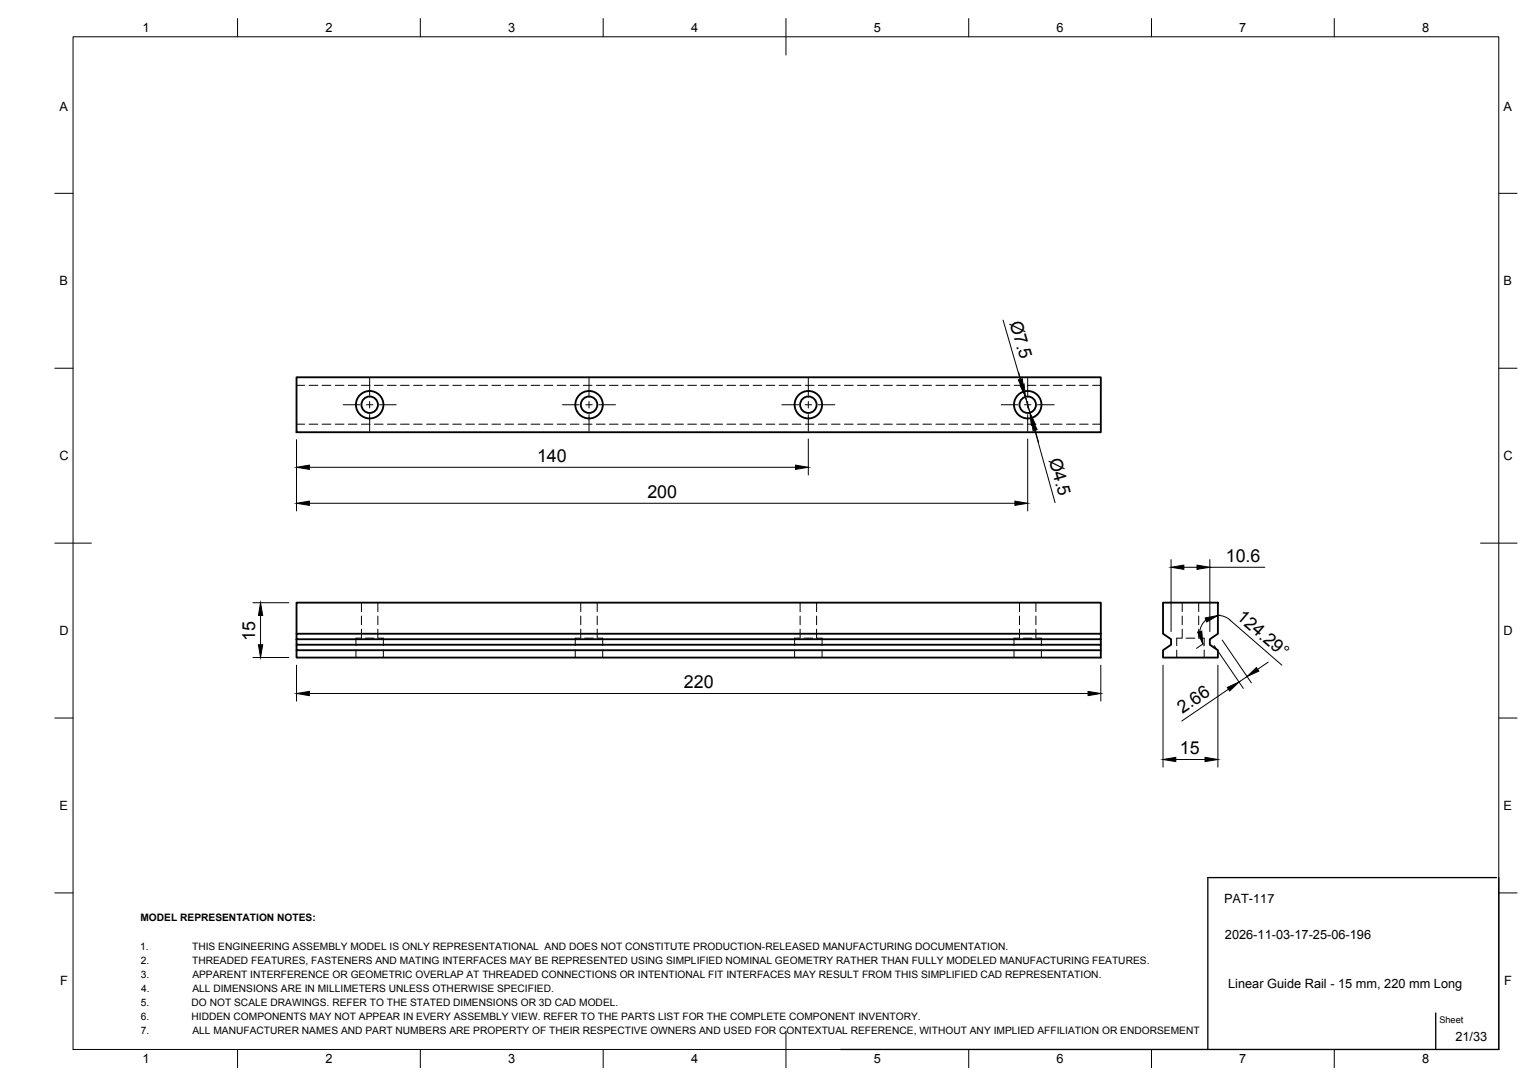
ISO-10303-21;
HEADER;
/* Generated by software containing ST-Developer
 * from STEP Tools, Inc. (www.steptools.com) 
 */

FILE_DESCRIPTION(
/* description */ ('Counterbalanced vertical column'),
/* implementation_level */ '2;1');

FILE_NAME(
/* name */ 'Linear Guide Rail - 15 mm, 220 mm Long.step',
/* time_stamp */ '2026-10-29T16:47:22-07:00',
/* author */ (''),
/* organization */ (''),
/* preprocessor_version */ 'ST-DEVELOPER v20.2',
/* originating_system */ 'Autodesk Translation Framework v15.17.0.0',
/* authorisation */ '');

FILE_SCHEMA (('AUTOMOTIVE_DESIGN { 1 0 10303 214 3 1 1 }'));
ENDSEC;

DATA;
#10=MECHANICAL_DESIGN_GEOMETRIC_PRESENTATION_REPRESENTATION('',(#368),#15040);
#298=SHAPE_REPRESENTATION_RELATIONSHIP('SRR','None',#15202,#333);
#333=ADVANCED_BREP_SHAPE_REPRESENTATION('',(#403),#15021);
#368=STYLED_ITEM('',(#15450),#403);
#403=MANIFOLD_SOLID_BREP('Body1',#7091);
#480=FACE_BOUND('',#1480,.T.);
#481=FACE_BOUND('',#1483,.T.);
#482=FACE_BOUND('',#1486,.T.);
#483=FACE_BOUND('',#1489,.T.);
#484=FACE_BOUND('',#1499,.T.);
#485=FACE_BOUND('',#1500,.T.);
#486=FACE_BOUND('',#1501,.T.);
#487=FACE_BOUND('',#1502,.T.);
#488=FACE_BOUND('',#1509,.T.);
#489=FACE_BOUND('',#1510,.T.);
#490=FACE_BOUND('',#1511,.T.);
#491=FACE_BOUND('',#1512,.T.);
#665=PLANE('',#7806);
#666=PLANE('',#7811);
#667=PLANE('',#7816);
#668=PLANE('',#7821);
#669=PLANE('',#7831);
#670=PLANE('',#7832);
#671=PLANE('',#7833);
#672=PLANE('',#7834);
#673=PLANE('',#7835);
#674=PLANE('',#7836);
#675=PLANE('',#7837);
#676=PLANE('',#7838);
#677=PLANE('',#7839);
#678=PLANE('',#7840);
#679=PLANE('',#7841);
#680=PLANE('',#7842);
#681=PLANE('',#7843);
#682=PLANE('',#7844);
#1009=FACE_OUTER_BOUND('',#1478,.T.);
#1010=FACE_OUTER_BOUND('',#1479,.T.);
#1011=FACE_OUTER_BOUND('',#1481,.T.);
#1012=FACE_OUTER_BOUND('',#1482,.T.);
#1013=FACE_OUTER_BOUND('',#1484,.T.);
#1014=FACE_OUTER_BOUND('',#1485,.T.);
#1015=FACE_OUTER_BOUND('',#1487,.T.);
#1016=FACE_OUTER_BOUND('',#1488,.T.);
#1017=FACE_OUTER_BOUND('',#1490,.T.);
#1018=FACE_OUTER_BOUND('',#1491,.T.);
#1019=FACE_OUTER_BOUND('',#1492,.T.);
#1020=FACE_OUTER_BOUND('',#1493,.T.);
#1021=FACE_OUTER_BOUND('',#1494,.T.);
#1022=FACE_OUTER_BOUND('',#1495,.T.);
#1023=FACE_OUTER_BOUND('',#1496,.T.);
#1024=FACE_OUTER_BOUND('',#1497,.T.);
#1025=FACE_OUTER_BOUND('',#1498,.T.);
#1026=FACE_OUTER_BOUND('',#1503,.T.);
#1027=FACE_OUTER_BOUND('',#1504,.T.);
#1028=FACE_OUTER_BOUND('',#1505,.T.);
#1029=FACE_OUTER_BOUND('',#1506,.T.);
#1030=FACE_OUTER_BOUND('',#1507,.T.);
#1031=FACE_OUTER_BOUND('',#1508,.T.);
#1032=FACE_OUTER_BOUND('',#1513,.T.);
#1033=FACE_OUTER_BOUND('',#1514,.T.);
#1034=FACE_OUTER_BOUND('',#1515,.T.);
#1478=EDGE_LOOP('',(#5586,#5587,#5588,#5589));
#1479=EDGE_LOOP('',(#5590));
#1480=EDGE_LOOP('',(#5591));
#1481=EDGE_LOOP('',(#5592,#5593,#5594,#5595));
#1482=EDGE_LOOP('',(#5596));
#1483=EDGE_LOOP('',(#5597));
#1484=EDGE_LOOP('',(#5598,#5599,#5600,#5601));
#1485=EDGE_LOOP('',(#5602));
#1486=EDGE_LOOP('',(#5603));
#1487=EDGE_LOOP('',(#5604,#5605,#5606,#5607));
#1488=EDGE_LOOP('',(#5608));
#1489=EDGE_LOOP('',(#5609));
#1490=EDGE_LOOP('',(#5610,#5611,#5612,#5613));
#1491=EDGE_LOOP('',(#5614,#5615,#5616,#5617));
#1492=EDGE_LOOP('',(#5618,#5619,#5620,#5621));
#1493=EDGE_LOOP('',(#5622,#5623,#5624,#5625));
#1494=EDGE_LOOP('',(#5626,#5627,#5628,#5629));
#1495=EDGE_LOOP('',(#5630,#5631,#5632,#5633));
#1496=EDGE_LOOP('',(#5634,#5635,#5636,#5637));
#1497=EDGE_LOOP('',(#5638,#5639,#5640,#5641));
#1498=EDGE_LOOP('',(#5642,#5643,#5644,#5645));
#1499=EDGE_LOOP('',(#5646));
#1500=EDGE_LOOP('',(#5647));
#1501=EDGE_LOOP('',(#5648));
#1502=EDGE_LOOP('',(#5649));
#1503=EDGE_LOOP('',(#5650,#5651,#5652,#5653));
#1504=EDGE_LOOP('',(#5654,#5655,#5656,#5657));
#1505=EDGE_LOOP('',(#5658,#5659,#5660,#5661));
#1506=EDGE_LOOP('',(#5662,#5663,#5664,#5665));
#1507=EDGE_LOOP('',(#5666,#5667,#5668,#5669));
#1508=EDGE_LOOP('',(#5670,#5671,#5672,#5673));
#1509=EDGE_LOOP('',(#5674));
#1510=EDGE_LOOP('',(#5675));
#1511=EDGE_LOOP('',(#5676));
#1512=EDGE_LOOP('',(#5677));
#1513=EDGE_LOOP('',(#5678,#5679,#5680,#5681));
#1514=EDGE_LOOP('',(#5682,#5683,#5684,#5685,#5686,#5687,#5688,#5689,#5690,
#5691,#5692,#5693));
#1515=EDGE_LOOP('',(#5694,#5695,#5696,#5697,#5698,#5699,#5700,#5701,#5702,
#5703,#5704,#5705));
#2047=LINE('',#13849,#2718);
#2048=LINE('',#13858,#2719);
#2049=LINE('',#13867,#2720);
#2050=LINE('',#13876,#2721);
#2051=LINE('',#13884,#2722);
#2052=LINE('',#13888,#2723);
#2053=LINE('',#13892,#2724);
#2054=LINE('',#13896,#2725);
#2055=LINE('',#13900,#2726);
#2056=LINE('',#13902,#2727);
#2057=LINE('',#13904,#2728);
#2058=LINE('',#13905,#2729);
#2059=LINE('',#13908,#2730);
#2060=LINE('',#13910,#2731);
#2061=LINE('',#13911,#2732);
#2062=LINE('',#13914,#2733);
#2063=LINE('',#13916,#2734);
#2064=LINE('',#13917,#2735);
#2065=LINE('',#13920,#2736);
#2066=LINE('',#13922,#2737);
#2067=LINE('',#13923,#2738);
#2068=LINE('',#13926,#2739);
#2069=LINE('',#13928,#2740);
#2070=LINE('',#13929,#2741);
#2071=LINE('',#13932,#2742);
#2072=LINE('',#13934,#2743);
#2073=LINE('',#13935,#2744);
#2074=LINE('',#13938,#2745);
#2075=LINE('',#13940,#2746);
#2076=LINE('',#13941,#2747);
#2077=LINE('',#13944,#2748);
#2078=LINE('',#13946,#2749);
#2079=LINE('',#13947,#2750);
#2080=LINE('',#13950,#2751);
#2081=LINE('',#13952,#2752);
#2082=LINE('',#13953,#2753);
#2083=LINE('',#13956,#2754);
#2084=LINE('',#13958,#2755);
#2085=LINE('',#13959,#2756);
#2086=LINE('',#13962,#2757);
#2087=LINE('',#13964,#2758);
#2088=LINE('',#13965,#2759);
#2089=LINE('',#13967,#2760);
#2090=LINE('',#13968,#2761);
#2718=VECTOR('',#9131,0.375);
#2719=VECTOR('',#9142,0.375);
#2720=VECTOR('',#9153,0.375);
#2721=VECTOR('',#9164,0.375);
#2722=VECTOR('',#9175,0.225);
#2723=VECTOR('',#9180,0.225);
#2724=VECTOR('',#9185,0.225);
#2725=VECTOR('',#9190,0.225000000000001);
#2726=VECTOR('',#9193,1.);
#2727=VECTOR('',#9194,1.);
#2728=VECTOR('',#9195,1.);
#2729=VECTOR('',#9196,1.);
#2730=VECTOR('',#9199,1.);
#2731=VECTOR('',#9200,1.);
#2732=VECTOR('',#9201,1.);
#2733=VECTOR('',#9204,1.);
#2734=VECTOR('',#9205,1.);
#2735=VECTOR('',#9206,1.);
#2736=VECTOR('',#9209,1.);
#2737=VECTOR('',#9210,1.);
#2738=VECTOR('',#9211,1.);
#2739=VECTOR('',#9214,1.);
#2740=VECTOR('',#9215,1.);
#2741=VECTOR('',#9216,1.);
#2742=VECTOR('',#9219,1.);
#2743=VECTOR('',#9220,1.);
#2744=VECTOR('',#9221,1.);
#2745=VECTOR('',#9224,1.);
#2746=VECTOR('',#9225,1.);
#2747=VECTOR('',#9226,1.);
#2748=VECTOR('',#9229,1.);
#2749=VECTOR('',#9230,1.);
#2750=VECTOR('',#9231,1.);
#2751=VECTOR('',#9234,1.);
#2752=VECTOR('',#9235,1.);
#2753=VECTOR('',#9236,1.);
#2754=VECTOR('',#9239,1.);
#2755=VECTOR('',#9240,1.);
#2756=VECTOR('',#9241,1.);
#2757=VECTOR('',#9244,1.);
#2758=VECTOR('',#9245,1.);
#2759=VECTOR('',#9246,1.);
#2760=VECTOR('',#9249,1.);
#2761=VECTOR('',#9250,1.);
#3189=CIRCLE('',#7804,0.375);
#3190=CIRCLE('',#7805,0.375);
#3191=CIRCLE('',#7807,0.225);
#3192=CIRCLE('',#7809,0.375);
#3193=CIRCLE('',#7810,0.375);
#3194=CIRCLE('',#7812,0.225);
#3195=CIRCLE('',#7814,0.375);
#3196=CIRCLE('',#7815,0.375);
#3197=CIRCLE('',#7817,0.225);
#3198=CIRCLE('',#7819,0.375);
#3199=CIRCLE('',#7820,0.375);
#3200=CIRCLE('',#7822,0.225000000000001);
#3201=CIRCLE('',#7824,0.225);
#3202=CIRCLE('',#7826,0.225);
#3203=CIRCLE('',#7828,0.225);
#3204=CIRCLE('',#7830,0.225000000000001);
#3572=VERTEX_POINT('',#13846);
#3573=VERTEX_POINT('',#13848);
#3574=VERTEX_POINT('',#13852);
#3575=VERTEX_POINT('',#13855);
#3576=VERTEX_POINT('',#13857);
#3577=VERTEX_POINT('',#13861);
#3578=VERTEX_POINT('',#13864);
#3579=VERTEX_POINT('',#13866);
#3580=VERTEX_POINT('',#13870);
#3581=VERTEX_POINT('',#13873);
#3582=VERTEX_POINT('',#13875);
#3583=VERTEX_POINT('',#13879);
#3584=VERTEX_POINT('',#13882);
#3585=VERTEX_POINT('',#13886);
#3586=VERTEX_POINT('',#13890);
#3587=VERTEX_POINT('',#13894);
#3588=VERTEX_POINT('',#13898);
#3589=VERTEX_POINT('',#13899);
#3590=VERTEX_POINT('',#13901);
#3591=VERTEX_POINT('',#13903);
#3592=VERTEX_POINT('',#13907);
#3593=VERTEX_POINT('',#13909);
#3594=VERTEX_POINT('',#13913);
#3595=VERTEX_POINT('',#13915);
#3596=VERTEX_POINT('',#13919);
#3597=VERTEX_POINT('',#13921);
#3598=VERTEX_POINT('',#13925);
#3599=VERTEX_POINT('',#13927);
#3600=VERTEX_POINT('',#13931);
#3601=VERTEX_POINT('',#13933);
#3602=VERTEX_POINT('',#13937);
#3603=VERTEX_POINT('',#13939);
#3604=VERTEX_POINT('',#13943);
#3605=VERTEX_POINT('',#13945);
#3606=VERTEX_POINT('',#13949);
#3607=VERTEX_POINT('',#13951);
#3608=VERTEX_POINT('',#13955);
#3609=VERTEX_POINT('',#13957);
#3610=VERTEX_POINT('',#13961);
#3611=VERTEX_POINT('',#13963);
#4294=EDGE_CURVE('',#3572,#3572,#3189,.T.);
#4295=EDGE_CURVE('',#3572,#3573,#2047,.T.);
#4296=EDGE_CURVE('',#3573,#3573,#3190,.T.);
#4297=EDGE_CURVE('',#3574,#3574,#3191,.T.);
#4298=EDGE_CURVE('',#3575,#3575,#3192,.T.);
#4299=EDGE_CURVE('',#3575,#3576,#2048,.T.);
#4300=EDGE_CURVE('',#3576,#3576,#3193,.T.);
#4301=EDGE_CURVE('',#3577,#3577,#3194,.T.);
#4302=EDGE_CURVE('',#3578,#3578,#3195,.T.);
#4303=EDGE_CURVE('',#3578,#3579,#2049,.T.);
#4304=EDGE_CURVE('',#3579,#3579,#3196,.T.);
#4305=EDGE_CURVE('',#3580,#3580,#3197,.T.);
#4306=EDGE_CURVE('',#3581,#3581,#3198,.T.);
#4307=EDGE_CURVE('',#3581,#3582,#2050,.T.);
#4308=EDGE_CURVE('',#3582,#3582,#3199,.T.);
#4309=EDGE_CURVE('',#3583,#3583,#3200,.T.);
#4310=EDGE_CURVE('',#3584,#3584,#3201,.T.);
#4311=EDGE_CURVE('',#3584,#3574,#2051,.T.);
#4312=EDGE_CURVE('',#3585,#3585,#3202,.T.);
#4313=EDGE_CURVE('',#3585,#3577,#2052,.T.);
#4314=EDGE_CURVE('',#3586,#3586,#3203,.T.);
#4315=EDGE_CURVE('',#3586,#3580,#2053,.T.);
#4316=EDGE_CURVE('',#3587,#3587,#3204,.T.);
#4317=EDGE_CURVE('',#3587,#3583,#2054,.T.);
#4318=EDGE_CURVE('',#3588,#3589,#2055,.T.);
#4319=EDGE_CURVE('',#3589,#3590,#2056,.T.);
#4320=EDGE_CURVE('',#3591,#3590,#2057,.T.);
#4321=EDGE_CURVE('',#3588,#3591,#2058,.T.);
#4322=EDGE_CURVE('',#3592,#3588,#2059,.T.);
#4323=EDGE_CURVE('',#3593,#3591,#2060,.T.);
#4324=EDGE_CURVE('',#3592,#3593,#2061,.T.);
#4325=EDGE_CURVE('',#3594,#3592,#2062,.T.);
#4326=EDGE_CURVE('',#3595,#3593,#2063,.T.);
#4327=EDGE_CURVE('',#3594,#3595,#2064,.T.);
#4328=EDGE_CURVE('',#3596,#3594,#2065,.T.);
#4329=EDGE_CURVE('',#3597,#3595,#2066,.T.);
#4330=EDGE_CURVE('',#3596,#3597,#2067,.T.);
#4331=EDGE_CURVE('',#3598,#3596,#2068,.T.);
#4332=EDGE_CURVE('',#3599,#3597,#2069,.T.);
#4333=EDGE_CURVE('',#3598,#3599,#2070,.T.);
#4334=EDGE_CURVE('',#3600,#3598,#2071,.T.);
#4335=EDGE_CURVE('',#3601,#3599,#2072,.T.);
#4336=EDGE_CURVE('',#3600,#3601,#2073,.T.);
#4337=EDGE_CURVE('',#3602,#3600,#2074,.T.);
#4338=EDGE_CURVE('',#3603,#3601,#2075,.T.);
#4339=EDGE_CURVE('',#3602,#3603,#2076,.T.);
#4340=EDGE_CURVE('',#3604,#3602,#2077,.T.);
#4341=EDGE_CURVE('',#3605,#3603,#2078,.T.);
#4342=EDGE_CURVE('',#3604,#3605,#2079,.T.);
#4343=EDGE_CURVE('',#3606,#3604,#2080,.T.);
#4344=EDGE_CURVE('',#3607,#3605,#2081,.T.);
#4345=EDGE_CURVE('',#3606,#3607,#2082,.T.);
#4346=EDGE_CURVE('',#3608,#3606,#2083,.T.);
#4347=EDGE_CURVE('',#3609,#3607,#2084,.T.);
#4348=EDGE_CURVE('',#3608,#3609,#2085,.T.);
#4349=EDGE_CURVE('',#3610,#3608,#2086,.T.);
#4350=EDGE_CURVE('',#3611,#3609,#2087,.T.);
#4351=EDGE_CURVE('',#3610,#3611,#2088,.T.);
#4352=EDGE_CURVE('',#3589,#3610,#2089,.T.);
#4353=EDGE_CURVE('',#3590,#3611,#2090,.T.);
#5586=ORIENTED_EDGE('',*,*,#4294,.F.);
#5587=ORIENTED_EDGE('',*,*,#4295,.T.);
#5588=ORIENTED_EDGE('',*,*,#4296,.F.);
#5589=ORIENTED_EDGE('',*,*,#4295,.F.);
#5590=ORIENTED_EDGE('',*,*,#4294,.T.);
#5591=ORIENTED_EDGE('',*,*,#4297,.F.);
#5592=ORIENTED_EDGE('',*,*,#4298,.F.);
#5593=ORIENTED_EDGE('',*,*,#4299,.T.);
#5594=ORIENTED_EDGE('',*,*,#4300,.F.);
#5595=ORIENTED_EDGE('',*,*,#4299,.F.);
#5596=ORIENTED_EDGE('',*,*,#4298,.T.);
#5597=ORIENTED_EDGE('',*,*,#4301,.F.);
#5598=ORIENTED_EDGE('',*,*,#4302,.F.);
#5599=ORIENTED_EDGE('',*,*,#4303,.T.);
#5600=ORIENTED_EDGE('',*,*,#4304,.F.);
#5601=ORIENTED_EDGE('',*,*,#4303,.F.);
#5602=ORIENTED_EDGE('',*,*,#4302,.T.);
#5603=ORIENTED_EDGE('',*,*,#4305,.F.);
#5604=ORIENTED_EDGE('',*,*,#4306,.F.);
#5605=ORIENTED_EDGE('',*,*,#4307,.T.);
#5606=ORIENTED_EDGE('',*,*,#4308,.F.);
#5607=ORIENTED_EDGE('',*,*,#4307,.F.);
#5608=ORIENTED_EDGE('',*,*,#4306,.T.);
#5609=ORIENTED_EDGE('',*,*,#4309,.F.);
#5610=ORIENTED_EDGE('',*,*,#4310,.F.);
#5611=ORIENTED_EDGE('',*,*,#4311,.T.);
#5612=ORIENTED_EDGE('',*,*,#4297,.T.);
#5613=ORIENTED_EDGE('',*,*,#4311,.F.);
#5614=ORIENTED_EDGE('',*,*,#4312,.F.);
#5615=ORIENTED_EDGE('',*,*,#4313,.T.);
#5616=ORIENTED_EDGE('',*,*,#4301,.T.);
#5617=ORIENTED_EDGE('',*,*,#4313,.F.);
#5618=ORIENTED_EDGE('',*,*,#4314,.F.);
#5619=ORIENTED_EDGE('',*,*,#4315,.T.);
#5620=ORIENTED_EDGE('',*,*,#4305,.T.);
#5621=ORIENTED_EDGE('',*,*,#4315,.F.);
#5622=ORIENTED_EDGE('',*,*,#4316,.F.);
#5623=ORIENTED_EDGE('',*,*,#4317,.T.);
#5624=ORIENTED_EDGE('',*,*,#4309,.T.);
#5625=ORIENTED_EDGE('',*,*,#4317,.F.);
#5626=ORIENTED_EDGE('',*,*,#4318,.T.);
#5627=ORIENTED_EDGE('',*,*,#4319,.T.);
#5628=ORIENTED_EDGE('',*,*,#4320,.F.);
#5629=ORIENTED_EDGE('',*,*,#4321,.F.);
#5630=ORIENTED_EDGE('',*,*,#4322,.T.);
#5631=ORIENTED_EDGE('',*,*,#4321,.T.);
#5632=ORIENTED_EDGE('',*,*,#4323,.F.);
#5633=ORIENTED_EDGE('',*,*,#4324,.F.);
#5634=ORIENTED_EDGE('',*,*,#4325,.T.);
#5635=ORIENTED_EDGE('',*,*,#4324,.T.);
#5636=ORIENTED_EDGE('',*,*,#4326,.F.);
#5637=ORIENTED_EDGE('',*,*,#4327,.F.);
#5638=ORIENTED_EDGE('',*,*,#4328,.T.);
#5639=ORIENTED_EDGE('',*,*,#4327,.T.);
#5640=ORIENTED_EDGE('',*,*,#4329,.F.);
#5641=ORIENTED_EDGE('',*,*,#4330,.F.);
#5642=ORIENTED_EDGE('',*,*,#4331,.T.);
#5643=ORIENTED_EDGE('',*,*,#4330,.T.);
#5644=ORIENTED_EDGE('',*,*,#4332,.F.);
#5645=ORIENTED_EDGE('',*,*,#4333,.F.);
#5646=ORIENTED_EDGE('',*,*,#4308,.T.);
#5647=ORIENTED_EDGE('',*,*,#4304,.T.);
#5648=ORIENTED_EDGE('',*,*,#4300,.T.);
#5649=ORIENTED_EDGE('',*,*,#4296,.T.);
#5650=ORIENTED_EDGE('',*,*,#4334,.T.);
#5651=ORIENTED_EDGE('',*,*,#4333,.T.);
#5652=ORIENTED_EDGE('',*,*,#4335,.F.);
#5653=ORIENTED_EDGE('',*,*,#4336,.F.);
#5654=ORIENTED_EDGE('',*,*,#4337,.T.);
#5655=ORIENTED_EDGE('',*,*,#4336,.T.);
#5656=ORIENTED_EDGE('',*,*,#4338,.F.);
#5657=ORIENTED_EDGE('',*,*,#4339,.F.);
#5658=ORIENTED_EDGE('',*,*,#4340,.T.);
#5659=ORIENTED_EDGE('',*,*,#4339,.T.);
#5660=ORIENTED_EDGE('',*,*,#4341,.F.);
#5661=ORIENTED_EDGE('',*,*,#4342,.F.);
#5662=ORIENTED_EDGE('',*,*,#4343,.T.);
#5663=ORIENTED_EDGE('',*,*,#4342,.T.);
#5664=ORIENTED_EDGE('',*,*,#4344,.F.);
#5665=ORIENTED_EDGE('',*,*,#4345,.F.);
#5666=ORIENTED_EDGE('',*,*,#4346,.T.);
#5667=ORIENTED_EDGE('',*,*,#4345,.T.);
#5668=ORIENTED_EDGE('',*,*,#4347,.F.);
#5669=ORIENTED_EDGE('',*,*,#4348,.F.);
#5670=ORIENTED_EDGE('',*,*,#4349,.T.);
#5671=ORIENTED_EDGE('',*,*,#4348,.T.);
#5672=ORIENTED_EDGE('',*,*,#4350,.F.);
#5673=ORIENTED_EDGE('',*,*,#4351,.F.);
#5674=ORIENTED_EDGE('',*,*,#4310,.T.);
#5675=ORIENTED_EDGE('',*,*,#4312,.T.);
#5676=ORIENTED_EDGE('',*,*,#4314,.T.);
#5677=ORIENTED_EDGE('',*,*,#4316,.T.);
#5678=ORIENTED_EDGE('',*,*,#4352,.T.);
#5679=ORIENTED_EDGE('',*,*,#4351,.T.);
#5680=ORIENTED_EDGE('',*,*,#4353,.F.);
#5681=ORIENTED_EDGE('',*,*,#4319,.F.);
#5682=ORIENTED_EDGE('',*,*,#4353,.T.);
#5683=ORIENTED_EDGE('',*,*,#4350,.T.);
#5684=ORIENTED_EDGE('',*,*,#4347,.T.);
#5685=ORIENTED_EDGE('',*,*,#4344,.T.);
#5686=ORIENTED_EDGE('',*,*,#4341,.T.);
#5687=ORIENTED_EDGE('',*,*,#4338,.T.);
#5688=ORIENTED_EDGE('',*,*,#4335,.T.);
#5689=ORIENTED_EDGE('',*,*,#4332,.T.);
#5690=ORIENTED_EDGE('',*,*,#4329,.T.);
#5691=ORIENTED_EDGE('',*,*,#4326,.T.);
#5692=ORIENTED_EDGE('',*,*,#4323,.T.);
#5693=ORIENTED_EDGE('',*,*,#4320,.T.);
#5694=ORIENTED_EDGE('',*,*,#4352,.F.);
#5695=ORIENTED_EDGE('',*,*,#4318,.F.);
#5696=ORIENTED_EDGE('',*,*,#4322,.F.);
#5697=ORIENTED_EDGE('',*,*,#4325,.F.);
#5698=ORIENTED_EDGE('',*,*,#4328,.F.);
#5699=ORIENTED_EDGE('',*,*,#4331,.F.);
#5700=ORIENTED_EDGE('',*,*,#4334,.F.);
#5701=ORIENTED_EDGE('',*,*,#4337,.F.);
#5702=ORIENTED_EDGE('',*,*,#4340,.F.);
#5703=ORIENTED_EDGE('',*,*,#4343,.F.);
#5704=ORIENTED_EDGE('',*,*,#4346,.F.);
#5705=ORIENTED_EDGE('',*,*,#4349,.F.);
#6622=CYLINDRICAL_SURFACE('',#7803,0.375);
#6623=CYLINDRICAL_SURFACE('',#7808,0.375);
#6624=CYLINDRICAL_SURFACE('',#7813,0.375);
#6625=CYLINDRICAL_SURFACE('',#7818,0.375);
#6626=CYLINDRICAL_SURFACE('',#7823,0.225);
#6627=CYLINDRICAL_SURFACE('',#7825,0.225);
#6628=CYLINDRICAL_SURFACE('',#7827,0.225);
#6629=CYLINDRICAL_SURFACE('',#7829,0.225000000000001);
#6851=ADVANCED_FACE('',(#1009),#6622,.F.);
#6852=ADVANCED_FACE('',(#1010,#480),#665,.T.);
#6853=ADVANCED_FACE('',(#1011),#6623,.F.);
#6854=ADVANCED_FACE('',(#1012,#481),#666,.T.);
#6855=ADVANCED_FACE('',(#1013),#6624,.F.);
#6856=ADVANCED_FACE('',(#1014,#482),#667,.T.);
#6857=ADVANCED_FACE('',(#1015),#6625,.F.);
#6858=ADVANCED_FACE('',(#1016,#483),#668,.T.);
#6859=ADVANCED_FACE('',(#1017),#6626,.F.);
#6860=ADVANCED_FACE('',(#1018),#6627,.F.);
#6861=ADVANCED_FACE('',(#1019),#6628,.F.);
#6862=ADVANCED_FACE('',(#1020),#6629,.F.);
#6863=ADVANCED_FACE('',(#1021),#669,.T.);
#6864=ADVANCED_FACE('',(#1022),#670,.T.);
#6865=ADVANCED_FACE('',(#1023),#671,.T.);
#6866=ADVANCED_FACE('',(#1024),#672,.T.);
#6867=ADVANCED_FACE('',(#1025,#484,#485,#486,#487),#673,.T.);
#6868=ADVANCED_FACE('',(#1026),#674,.T.);
#6869=ADVANCED_FACE('',(#1027),#675,.T.);
#6870=ADVANCED_FACE('',(#1028),#676,.T.);
#6871=ADVANCED_FACE('',(#1029),#677,.T.);
#6872=ADVANCED_FACE('',(#1030),#678,.T.);
#6873=ADVANCED_FACE('',(#1031,#488,#489,#490,#491),#679,.T.);
#6874=ADVANCED_FACE('',(#1032),#680,.T.);
#6875=ADVANCED_FACE('',(#1033),#681,.T.);
#6876=ADVANCED_FACE('',(#1034),#682,.F.);
#7091=CLOSED_SHELL('',(#6851,#6852,#6853,#6854,#6855,#6856,#6857,#6858,
#6859,#6860,#6861,#6862,#6863,#6864,#6865,#6866,#6867,#6868,#6869,#6870,
#6871,#6872,#6873,#6874,#6875,#6876));
#7802=AXIS2_PLACEMENT_3D('',#13844,#9125,#9126);
#7803=AXIS2_PLACEMENT_3D('',#13845,#9127,#9128);
#7804=AXIS2_PLACEMENT_3D('',#13847,#9129,#9130);
#7805=AXIS2_PLACEMENT_3D('',#13850,#9132,#9133);
#7806=AXIS2_PLACEMENT_3D('',#13851,#9134,#9135);
#7807=AXIS2_PLACEMENT_3D('',#13853,#9136,#9137);
#7808=AXIS2_PLACEMENT_3D('',#13854,#9138,#9139);
#7809=AXIS2_PLACEMENT_3D('',#13856,#9140,#9141);
#7810=AXIS2_PLACEMENT_3D('',#13859,#9143,#9144);
#7811=AXIS2_PLACEMENT_3D('',#13860,#9145,#9146);
#7812=AXIS2_PLACEMENT_3D('',#13862,#9147,#9148);
#7813=AXIS2_PLACEMENT_3D('',#13863,#9149,#9150);
#7814=AXIS2_PLACEMENT_3D('',#13865,#9151,#9152);
#7815=AXIS2_PLACEMENT_3D('',#13868,#9154,#9155);
#7816=AXIS2_PLACEMENT_3D('',#13869,#9156,#9157);
#7817=AXIS2_PLACEMENT_3D('',#13871,#9158,#9159);
#7818=AXIS2_PLACEMENT_3D('',#13872,#9160,#9161);
#7819=AXIS2_PLACEMENT_3D('',#13874,#9162,#9163);
#7820=AXIS2_PLACEMENT_3D('',#13877,#9165,#9166);
#7821=AXIS2_PLACEMENT_3D('',#13878,#9167,#9168);
#7822=AXIS2_PLACEMENT_3D('',#13880,#9169,#9170);
#7823=AXIS2_PLACEMENT_3D('',#13881,#9171,#9172);
#7824=AXIS2_PLACEMENT_3D('',#13883,#9173,#9174);
#7825=AXIS2_PLACEMENT_3D('',#13885,#9176,#9177);
#7826=AXIS2_PLACEMENT_3D('',#13887,#9178,#9179);
#7827=AXIS2_PLACEMENT_3D('',#13889,#9181,#9182);
#7828=AXIS2_PLACEMENT_3D('',#13891,#9183,#9184);
#7829=AXIS2_PLACEMENT_3D('',#13893,#9186,#9187);
#7830=AXIS2_PLACEMENT_3D('',#13895,#9188,#9189);
#7831=AXIS2_PLACEMENT_3D('',#13897,#9191,#9192);
#7832=AXIS2_PLACEMENT_3D('',#13906,#9197,#9198);
#7833=AXIS2_PLACEMENT_3D('',#13912,#9202,#9203);
#7834=AXIS2_PLACEMENT_3D('',#13918,#9207,#9208);
#7835=AXIS2_PLACEMENT_3D('',#13924,#9212,#9213);
#7836=AXIS2_PLACEMENT_3D('',#13930,#9217,#9218);
#7837=AXIS2_PLACEMENT_3D('',#13936,#9222,#9223);
#7838=AXIS2_PLACEMENT_3D('',#13942,#9227,#9228);
#7839=AXIS2_PLACEMENT_3D('',#13948,#9232,#9233);
#7840=AXIS2_PLACEMENT_3D('',#13954,#9237,#9238);
#7841=AXIS2_PLACEMENT_3D('',#13960,#9242,#9243);
#7842=AXIS2_PLACEMENT_3D('',#13966,#9247,#9248);
#7843=AXIS2_PLACEMENT_3D('',#13969,#9251,#9252);
#7844=AXIS2_PLACEMENT_3D('',#13970,#9253,#9254);
#9125=DIRECTION('axis',(0.,0.,1.));
#9126=DIRECTION('refdir',(1.,0.,0.));
#9127=DIRECTION('center_axis',(0.,0.,1.));
#9128=DIRECTION('ref_axis',(1.,0.,0.));
#9129=DIRECTION('center_axis',(0.,0.,1.));
#9130=DIRECTION('ref_axis',(1.,0.,0.));
#9131=DIRECTION('',(0.,0.,1.));
#9132=DIRECTION('center_axis',(0.,0.,-1.));
#9133=DIRECTION('ref_axis',(1.,0.,0.));
#9134=DIRECTION('center_axis',(0.,0.,1.));
#9135=DIRECTION('ref_axis',(1.,0.,0.));
#9136=DIRECTION('center_axis',(0.,0.,1.));
#9137=DIRECTION('ref_axis',(1.,0.,0.));
#9138=DIRECTION('center_axis',(0.,0.,1.));
#9139=DIRECTION('ref_axis',(1.,0.,0.));
#9140=DIRECTION('center_axis',(0.,0.,1.));
#9141=DIRECTION('ref_axis',(1.,0.,0.));
#9142=DIRECTION('',(0.,0.,1.));
#9143=DIRECTION('center_axis',(0.,0.,-1.));
#9144=DIRECTION('ref_axis',(1.,0.,0.));
#9145=DIRECTION('center_axis',(0.,0.,1.));
#9146=DIRECTION('ref_axis',(1.,0.,0.));
#9147=DIRECTION('center_axis',(0.,0.,1.));
#9148=DIRECTION('ref_axis',(1.,0.,0.));
#9149=DIRECTION('center_axis',(0.,0.,1.));
#9150=DIRECTION('ref_axis',(1.,0.,0.));
#9151=DIRECTION('center_axis',(0.,0.,1.));
#9152=DIRECTION('ref_axis',(1.,0.,0.));
#9153=DIRECTION('',(0.,0.,1.));
#9154=DIRECTION('center_axis',(0.,0.,-1.));
#9155=DIRECTION('ref_axis',(1.,0.,0.));
#9156=DIRECTION('center_axis',(0.,0.,1.));
#9157=DIRECTION('ref_axis',(1.,0.,0.));
#9158=DIRECTION('center_axis',(0.,0.,1.));
#9159=DIRECTION('ref_axis',(1.,0.,0.));
#9160=DIRECTION('center_axis',(0.,0.,1.));
#9161=DIRECTION('ref_axis',(1.,0.,0.));
#9162=DIRECTION('center_axis',(0.,0.,1.));
#9163=DIRECTION('ref_axis',(1.,0.,0.));
#9164=DIRECTION('',(0.,0.,1.));
#9165=DIRECTION('center_axis',(0.,0.,-1.));
#9166=DIRECTION('ref_axis',(1.,0.,0.));
#9167=DIRECTION('center_axis',(0.,0.,1.));
#9168=DIRECTION('ref_axis',(1.,0.,0.));
#9169=DIRECTION('center_axis',(0.,0.,1.));
#9170=DIRECTION('ref_axis',(1.,0.,0.));
#9171=DIRECTION('center_axis',(0.,0.,1.));
#9172=DIRECTION('ref_axis',(1.,0.,0.));
#9173=DIRECTION('center_axis',(0.,0.,1.));
#9174=DIRECTION('ref_axis',(1.,0.,0.));
#9175=DIRECTION('',(0.,0.,1.));
#9176=DIRECTION('center_axis',(0.,0.,1.));
#9177=DIRECTION('ref_axis',(1.,0.,0.));
#9178=DIRECTION('center_axis',(0.,0.,1.));
#9179=DIRECTION('ref_axis',(1.,0.,0.));
#9180=DIRECTION('',(0.,0.,1.));
#9181=DIRECTION('center_axis',(0.,0.,1.));
#9182=DIRECTION('ref_axis',(1.,0.,0.));
#9183=DIRECTION('center_axis',(0.,0.,1.));
#9184=DIRECTION('ref_axis',(1.,0.,0.));
#9185=DIRECTION('',(0.,0.,1.));
#9186=DIRECTION('center_axis',(0.,0.,1.));
#9187=DIRECTION('ref_axis',(1.,0.,0.));
#9188=DIRECTION('center_axis',(0.,0.,1.));
#9189=DIRECTION('ref_axis',(1.,0.,0.));
#9190=DIRECTION('',(0.,0.,1.));
#9191=DIRECTION('center_axis',(0.,-0.56333682464151,0.826227342807548));
#9192=DIRECTION('ref_axis',(0.,-0.826227342807548,-0.56333682464151));
#9193=DIRECTION('',(0.,-0.826227342807548,-0.56333682464151));
#9194=DIRECTION('',(1.,0.,0.));
#9195=DIRECTION('',(0.,-0.826227342807548,-0.56333682464151));
#9196=DIRECTION('',(1.,0.,0.));
#9197=DIRECTION('center_axis',(0.,-1.,0.));
#9198=DIRECTION('ref_axis',(0.,0.,-1.));
#9199=DIRECTION('',(0.,0.,-1.));
#9200=DIRECTION('',(0.,0.,-1.));
#9201=DIRECTION('',(1.,0.,0.));
#9202=DIRECTION('center_axis',(0.,-0.56333682464151,-0.826227342807548));
#9203=DIRECTION('ref_axis',(0.,0.826227342807548,-0.56333682464151));
#9204=DIRECTION('',(0.,0.826227342807548,-0.56333682464151));
#9205=DIRECTION('',(0.,0.826227342807548,-0.56333682464151));
#9206=DIRECTION('',(1.,0.,0.));
#9207=DIRECTION('center_axis',(0.,-1.,0.));
#9208=DIRECTION('ref_axis',(0.,0.,-1.));
#9209=DIRECTION('',(0.,0.,-1.));
#9210=DIRECTION('',(0.,0.,-1.));
#9211=DIRECTION('',(1.,0.,0.));
#9212=DIRECTION('center_axis',(0.,0.,1.));
#9213=DIRECTION('ref_axis',(0.,-1.,0.));
#9214=DIRECTION('',(0.,-1.,0.));
#9215=DIRECTION('',(0.,-1.,0.));
#9216=DIRECTION('',(1.,0.,0.));
#9217=DIRECTION('center_axis',(0.,1.,0.));
#9218=DIRECTION('ref_axis',(0.,0.,1.));
#9219=DIRECTION('',(0.,0.,1.));
#9220=DIRECTION('',(0.,0.,1.));
#9221=DIRECTION('',(1.,0.,0.));
#9222=DIRECTION('center_axis',(0.,0.56333682464151,-0.826227342807548));
#9223=DIRECTION('ref_axis',(0.,0.826227342807548,0.56333682464151));
#9224=DIRECTION('',(0.,0.826227342807548,0.56333682464151));
#9225=DIRECTION('',(0.,0.826227342807548,0.56333682464151));
#9226=DIRECTION('',(1.,0.,0.));
#9227=DIRECTION('center_axis',(0.,1.,0.));
#9228=DIRECTION('ref_axis',(0.,0.,1.));
#9229=DIRECTION('',(0.,0.,1.));
#9230=DIRECTION('',(0.,0.,1.));
#9231=DIRECTION('',(1.,0.,0.));
#9232=DIRECTION('center_axis',(0.,0.56333682464151,0.826227342807548));
#9233=DIRECTION('ref_axis',(0.,-0.826227342807548,0.56333682464151));
#9234=DIRECTION('',(0.,-0.826227342807548,0.56333682464151));
#9235=DIRECTION('',(0.,-0.826227342807548,0.56333682464151));
#9236=DIRECTION('',(1.,0.,0.));
#9237=DIRECTION('center_axis',(0.,1.,0.));
#9238=DIRECTION('ref_axis',(0.,0.,1.));
#9239=DIRECTION('',(0.,0.,1.));
#9240=DIRECTION('',(0.,0.,1.));
#9241=DIRECTION('',(1.,0.,0.));
#9242=DIRECTION('center_axis',(0.,0.,-1.));
#9243=DIRECTION('ref_axis',(0.,1.,0.));
#9244=DIRECTION('',(0.,1.,0.));
#9245=DIRECTION('',(0.,1.,0.));
#9246=DIRECTION('',(1.,0.,0.));
#9247=DIRECTION('center_axis',(0.,-1.,0.));
#9248=DIRECTION('ref_axis',(0.,0.,-1.));
#9249=DIRECTION('',(0.,0.,-1.));
#9250=DIRECTION('',(0.,0.,-1.));
#9251=DIRECTION('center_axis',(1.,0.,0.));
#9252=DIRECTION('ref_axis',(0.,0.,-1.));
#9253=DIRECTION('center_axis',(1.,0.,0.));
#9254=DIRECTION('ref_axis',(0.,0.,-1.));
#13844=CARTESIAN_POINT('',(0.,0.,0.));
#13845=CARTESIAN_POINT('Origin',(14.,0.,0.97));
#13846=CARTESIAN_POINT('',(13.625,-4.59242549680257E-17,0.97));
#13847=CARTESIAN_POINT('Origin',(14.,0.,0.97));
#13848=CARTESIAN_POINT('',(13.625,4.59242549680257E-17,1.5));
#13849=CARTESIAN_POINT('',(13.625,-4.59242549680257E-17,0.97));
#13850=CARTESIAN_POINT('Origin',(14.,0.,1.5));
#13851=CARTESIAN_POINT('Origin',(14.,0.,0.97));
#13852=CARTESIAN_POINT('',(13.775,-2.75545529808154E-17,0.97));
#13853=CARTESIAN_POINT('Origin',(14.,0.,0.97));
#13854=CARTESIAN_POINT('Origin',(8.,0.,0.97));
#13855=CARTESIAN_POINT('',(7.625,-4.59242549680257E-17,0.97));
#13856=CARTESIAN_POINT('Origin',(8.,0.,0.97));
#13857=CARTESIAN_POINT('',(7.625,4.59242549680257E-17,1.5));
#13858=CARTESIAN_POINT('',(7.625,-4.59242549680257E-17,0.97));
#13859=CARTESIAN_POINT('Origin',(8.,0.,1.5));
#13860=CARTESIAN_POINT('Origin',(8.,0.,0.97));
#13861=CARTESIAN_POINT('',(7.775,-2.75545529808154E-17,0.97));
#13862=CARTESIAN_POINT('Origin',(8.,0.,0.97));
#13863=CARTESIAN_POINT('Origin',(2.,0.,0.97));
#13864=CARTESIAN_POINT('',(1.625,-4.59242549680257E-17,0.97));
#13865=CARTESIAN_POINT('Origin',(2.,0.,0.97));
#13866=CARTESIAN_POINT('',(1.625,4.59242549680257E-17,1.5));
#13867=CARTESIAN_POINT('',(1.625,-4.59242549680257E-17,0.97));
#13868=CARTESIAN_POINT('Origin',(2.,0.,1.5));
#13869=CARTESIAN_POINT('Origin',(2.,0.,0.97));
#13870=CARTESIAN_POINT('',(1.775,-2.75545529808155E-17,0.97));
#13871=CARTESIAN_POINT('Origin',(2.,0.,0.97));
#13872=CARTESIAN_POINT('Origin',(20.,0.,0.97));
#13873=CARTESIAN_POINT('',(19.625,-4.59242549680257E-17,0.97));
#13874=CARTESIAN_POINT('Origin',(20.,0.,0.97));
#13875=CARTESIAN_POINT('',(19.625,4.59242549680257E-17,1.5));
#13876=CARTESIAN_POINT('',(19.625,-4.59242549680257E-17,0.97));
#13877=CARTESIAN_POINT('Origin',(20.,0.,1.5));
#13878=CARTESIAN_POINT('Origin',(20.,0.,0.97));
#13879=CARTESIAN_POINT('',(19.775,-2.75545529808156E-17,0.97));
#13880=CARTESIAN_POINT('Origin',(20.,0.,0.97));
#13881=CARTESIAN_POINT('Origin',(14.,0.,-0.1));
#13882=CARTESIAN_POINT('',(13.775,-2.75545529808154E-17,0.));
#13883=CARTESIAN_POINT('Origin',(14.,0.,0.));
#13884=CARTESIAN_POINT('',(13.775,-2.75545529808154E-17,-0.1));
#13885=CARTESIAN_POINT('Origin',(8.,0.,-0.1));
#13886=CARTESIAN_POINT('',(7.775,-2.75545529808154E-17,0.));
#13887=CARTESIAN_POINT('Origin',(8.,0.,0.));
#13888=CARTESIAN_POINT('',(7.775,-2.75545529808154E-17,-0.1));
#13889=CARTESIAN_POINT('Origin',(2.,0.,-0.1));
#13890=CARTESIAN_POINT('',(1.775,-2.75545529808155E-17,0.));
#13891=CARTESIAN_POINT('Origin',(2.,0.,0.));
#13892=CARTESIAN_POINT('',(1.775,-2.75545529808155E-17,-0.1));
#13893=CARTESIAN_POINT('Origin',(20.,0.,-0.1));
#13894=CARTESIAN_POINT('',(19.775,-2.75545529808156E-17,0.));
#13895=CARTESIAN_POINT('Origin',(20.,0.,0.));
#13896=CARTESIAN_POINT('',(19.775,-2.75545529808156E-17,-0.1));
#13897=CARTESIAN_POINT('Origin',(0.,-0.53,1.));
#13898=CARTESIAN_POINT('',(0.,-0.53,1.));
#13899=CARTESIAN_POINT('',(0.,-0.75,0.85));
#13900=CARTESIAN_POINT('',(0.,-0.53,1.));
#13901=CARTESIAN_POINT('',(22.,-0.75,0.85));
#13902=CARTESIAN_POINT('',(0.,-0.75,0.85));
#13903=CARTESIAN_POINT('',(22.,-0.53,1.));
#13904=CARTESIAN_POINT('',(22.,-0.53,1.));
#13905=CARTESIAN_POINT('',(0.,-0.53,1.));
#13906=CARTESIAN_POINT('Origin',(0.,-0.53,1.15));
#13907=CARTESIAN_POINT('',(0.,-0.53,1.15));
#13908=CARTESIAN_POINT('',(0.,-0.53,1.15));
#13909=CARTESIAN_POINT('',(22.,-0.53,1.15));
#13910=CARTESIAN_POINT('',(22.,-0.53,1.15));
#13911=CARTESIAN_POINT('',(0.,-0.53,1.15));
#13912=CARTESIAN_POINT('Origin',(0.,-0.75,1.3));
#13913=CARTESIAN_POINT('',(0.,-0.75,1.3));
#13914=CARTESIAN_POINT('',(0.,-0.75,1.3));
#13915=CARTESIAN_POINT('',(22.,-0.75,1.3));
#13916=CARTESIAN_POINT('',(22.,-0.75,1.3));
#13917=CARTESIAN_POINT('',(0.,-0.75,1.3));
#13918=CARTESIAN_POINT('Origin',(0.,-0.75,1.5));
#13919=CARTESIAN_POINT('',(0.,-0.75,1.5));
#13920=CARTESIAN_POINT('',(0.,-0.75,1.5));
#13921=CARTESIAN_POINT('',(22.,-0.75,1.5));
#13922=CARTESIAN_POINT('',(22.,-0.75,1.5));
#13923=CARTESIAN_POINT('',(0.,-0.75,1.5));
#13924=CARTESIAN_POINT('Origin',(0.,0.75,1.5));
#13925=CARTESIAN_POINT('',(0.,0.75,1.5));
#13926=CARTESIAN_POINT('',(0.,0.75,1.5));
#13927=CARTESIAN_POINT('',(22.,0.75,1.5));
#13928=CARTESIAN_POINT('',(22.,0.75,1.5));
#13929=CARTESIAN_POINT('',(0.,0.75,1.5));
#13930=CARTESIAN_POINT('Origin',(0.,0.75,1.3));
#13931=CARTESIAN_POINT('',(0.,0.75,1.3));
#13932=CARTESIAN_POINT('',(0.,0.75,1.3));
#13933=CARTESIAN_POINT('',(22.,0.75,1.3));
#13934=CARTESIAN_POINT('',(22.,0.75,1.3));
#13935=CARTESIAN_POINT('',(0.,0.75,1.3));
#13936=CARTESIAN_POINT('Origin',(0.,0.53,1.15));
#13937=CARTESIAN_POINT('',(0.,0.53,1.15));
#13938=CARTESIAN_POINT('',(0.,0.53,1.15));
#13939=CARTESIAN_POINT('',(22.,0.53,1.15));
#13940=CARTESIAN_POINT('',(22.,0.53,1.15));
#13941=CARTESIAN_POINT('',(0.,0.53,1.15));
#13942=CARTESIAN_POINT('Origin',(0.,0.53,1.));
#13943=CARTESIAN_POINT('',(0.,0.53,1.));
#13944=CARTESIAN_POINT('',(0.,0.53,1.));
#13945=CARTESIAN_POINT('',(22.,0.53,1.));
#13946=CARTESIAN_POINT('',(22.,0.53,1.));
#13947=CARTESIAN_POINT('',(0.,0.53,1.));
#13948=CARTESIAN_POINT('Origin',(0.,0.75,0.85));
#13949=CARTESIAN_POINT('',(0.,0.75,0.85));
#13950=CARTESIAN_POINT('',(0.,0.75,0.85));
#13951=CARTESIAN_POINT('',(22.,0.75,0.85));
#13952=CARTESIAN_POINT('',(22.,0.75,0.85));
#13953=CARTESIAN_POINT('',(0.,0.75,0.85));
#13954=CARTESIAN_POINT('Origin',(0.,0.75,0.));
#13955=CARTESIAN_POINT('',(0.,0.75,0.));
#13956=CARTESIAN_POINT('',(0.,0.75,0.));
#13957=CARTESIAN_POINT('',(22.,0.75,0.));
#13958=CARTESIAN_POINT('',(22.,0.75,0.));
#13959=CARTESIAN_POINT('',(0.,0.75,0.));
#13960=CARTESIAN_POINT('Origin',(0.,-0.75,0.));
#13961=CARTESIAN_POINT('',(0.,-0.75,0.));
#13962=CARTESIAN_POINT('',(0.,-0.75,0.));
#13963=CARTESIAN_POINT('',(22.,-0.75,0.));
#13964=CARTESIAN_POINT('',(22.,-0.75,0.));
#13965=CARTESIAN_POINT('',(0.,-0.75,0.));
#13966=CARTESIAN_POINT('Origin',(0.,-0.75,0.85));
#13967=CARTESIAN_POINT('',(0.,-0.75,0.85));
#13968=CARTESIAN_POINT('',(22.,-0.75,0.85));
#13969=CARTESIAN_POINT('Origin',(22.,0.,0.75));
#13970=CARTESIAN_POINT('Origin',(0.,0.,0.75));
#14981=UNCERTAINTY_MEASURE_WITH_UNIT(LENGTH_MEASURE(0.001),#15041,
'DISTANCE_ACCURACY_VALUE',
'Maximum model space distance between geometric entities at asserted c
onnectivities');
#15000=UNCERTAINTY_MEASURE_WITH_UNIT(LENGTH_MEASURE(0.001),#15041,
'DISTANCE_ACCURACY_VALUE',
'Maximum model space distance between geometric entities at asserted c
onnectivities');
#15021=(
GEOMETRIC_REPRESENTATION_CONTEXT(3)
GLOBAL_UNCERTAINTY_ASSIGNED_CONTEXT((#14981))
GLOBAL_UNIT_ASSIGNED_CONTEXT((#15041,#15043,#15044))
REPRESENTATION_CONTEXT('','3D')
);
#15040=(
GEOMETRIC_REPRESENTATION_CONTEXT(3)
GLOBAL_UNCERTAINTY_ASSIGNED_CONTEXT((#15000))
GLOBAL_UNIT_ASSIGNED_CONTEXT((#15041,#15043,#15044))
REPRESENTATION_CONTEXT('','3D')
);
#15041=(
LENGTH_UNIT()
NAMED_UNIT(*)
SI_UNIT(.CENTI.,.METRE.)
);
#15043=(
NAMED_UNIT(*)
PLANE_ANGLE_UNIT()
SI_UNIT($,.RADIAN.)
);
#15044=(
NAMED_UNIT(*)
SI_UNIT($,.STERADIAN.)
SOLID_ANGLE_UNIT()
);
#15065=SHAPE_DEFINITION_REPRESENTATION(#15104,#15202);
#15104=PRODUCT_DEFINITION_SHAPE('',$,#15242);
#15202=SHAPE_REPRESENTATION('',(#7802),#15021);
#15221=PRODUCT_DEFINITION_CONTEXT('part definition',#15340,'design');
#15242=PRODUCT_DEFINITION('Linear Guide Rail - 15 mm, 220 mm Long',
'Linear Guide Rail - 15 mm, 220 mm Long',#15281,#15221);
#15281=PRODUCT_DEFINITION_FORMATION('',$,#15362);
#15340=APPLICATION_CONTEXT(
'Core Data for Automotive Mechanical Design Process');
#15341=PRODUCT_CONTEXT('part definition',#15340,'mechanical');
#15362=PRODUCT('Linear Guide Rail - 15 mm, 220 mm Long',
'Linear Guide Rail - 15 mm, 220 mm Long',
'Linear Guide Rail - 15 mm, 220 mm Long',(#15341));
#15444=COLOUR_RGB('Sky Blue',0.24,0.69,0.87);
#15445=FILL_AREA_STYLE_COLOUR('',#15444);
#15446=FILL_AREA_STYLE('',(#15445));
#15447=SURFACE_STYLE_FILL_AREA(#15446);
#15448=SURFACE_SIDE_STYLE('',(#15447));
#15449=SURFACE_STYLE_USAGE(.BOTH.,#15448);
#15450=PRESENTATION_STYLE_ASSIGNMENT((#15449));
ENDSEC;
END-ISO-10303-21;
